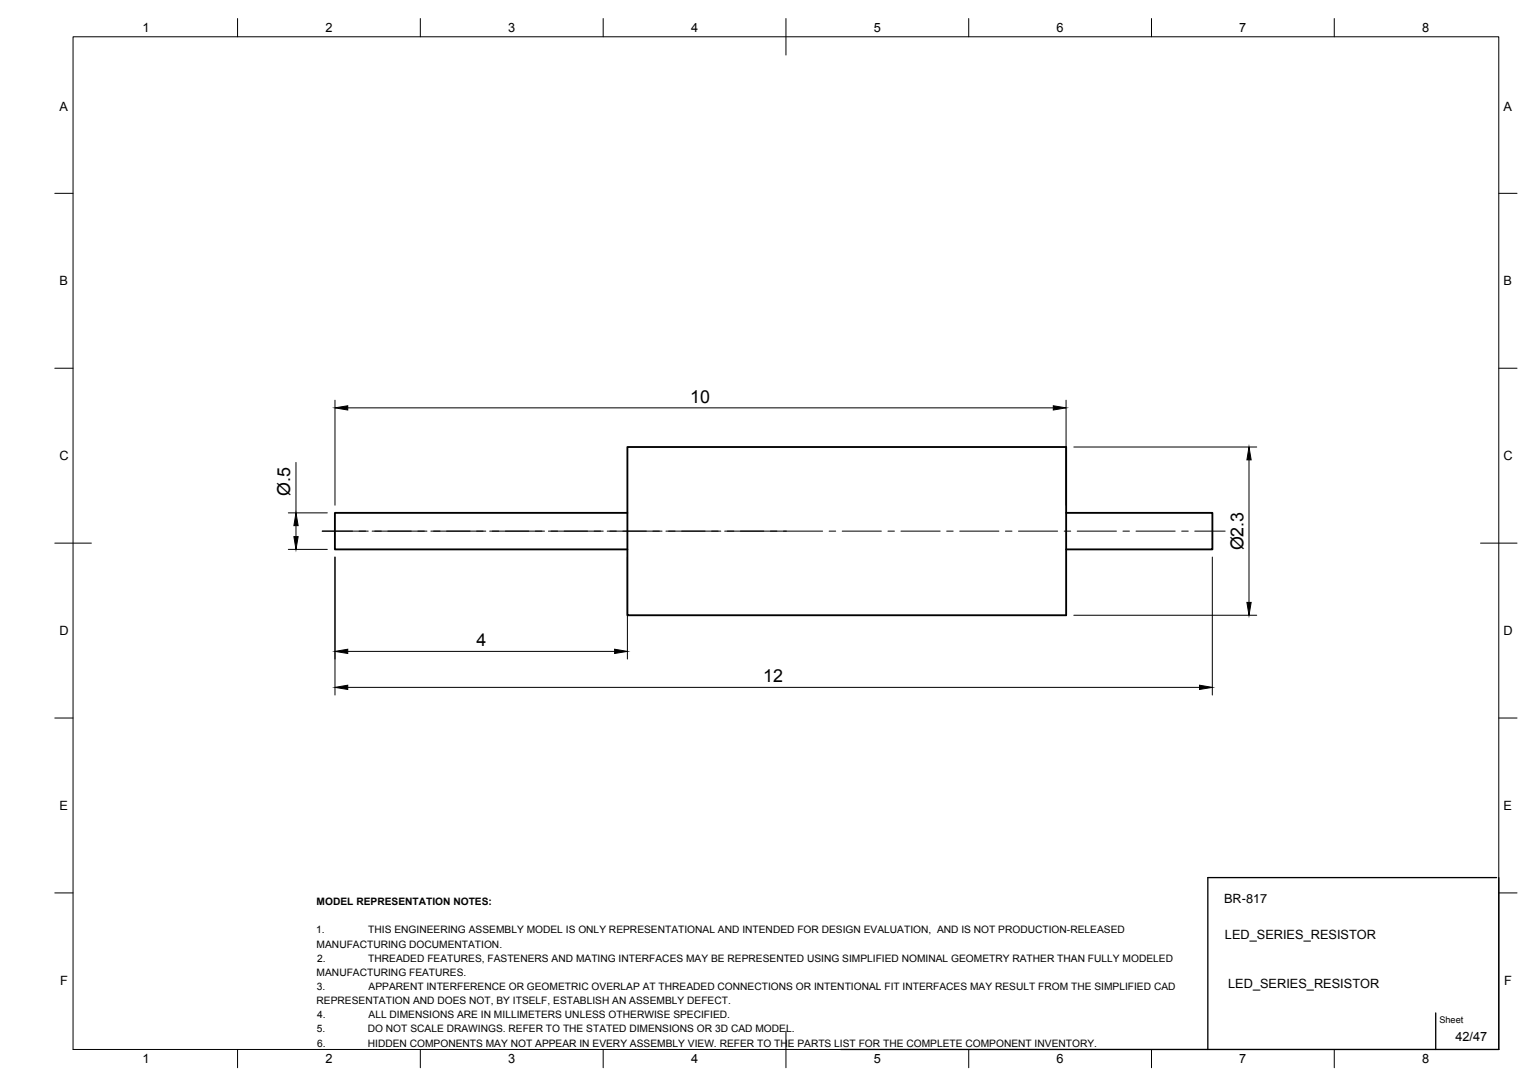
ISO-10303-21;
HEADER;
FILE_DESCRIPTION((''),'2;1');
FILE_NAME('LED_SERIES_RESISTOR.step','2026-10-01T22:07:29-07:00',(''),(''),'','','');
FILE_SCHEMA (('AUTOMOTIVE_DESIGN { 1 0 10303 214 3 1 1 }'));
ENDSEC;
DATA;
#10=MECHANICAL_DESIGN_GEOMETRIC_PRESENTATION_REPRESENTATION('',(#575,#576,#577),#15484);
#502=SHAPE_REPRESENTATION_RELATIONSHIP('SRR','None',#15653,#537) ;
#537=ADVANCED_BREP_SHAPE_REPRESENTATION('',(#616,#617,#618),#15477) ;
#575=STYLED_ITEM('',(#15833),#616) ;
#576=STYLED_ITEM('',(#15842),#617) ;
#577=STYLED_ITEM('',(#15842),#618) ;
#616=MANIFOLD_SOLID_BREP('RESISTOR_BODY',#8286) ;
#617=MANIFOLD_SOLID_BREP('RESISTOR_LEADS',#8287) ;
#618=MANIFOLD_SOLID_BREP('RESISTOR_LEADS',#8288) ;
#798=CYLINDRICAL_SURFACE('',#9829,0.115) ;
#799=CYLINDRICAL_SURFACE('',#9834,0.025) ;
#800=CYLINDRICAL_SURFACE('',#9839,0.025) ;
#1337=CIRCLE('',#9830,0.115) ;
#1338=CIRCLE('',#9831,0.115) ;
#1339=CIRCLE('',#9835,0.025) ;
#1340=CIRCLE('',#9836,0.025) ;
#1341=CIRCLE('',#9840,0.025) ;
#1342=CIRCLE('',#9841,0.025) ;
#1822=FACE_OUTER_BOUND('',#2393,.T.) ;
#1823=FACE_OUTER_BOUND('',#2394,.T.) ;
#1824=FACE_OUTER_BOUND('',#2395,.T.) ;
#1825=FACE_OUTER_BOUND('',#2396,.T.) ;
#1826=FACE_OUTER_BOUND('',#2397,.T.) ;
#1827=FACE_OUTER_BOUND('',#2398,.T.) ;
#1828=FACE_OUTER_BOUND('',#2399,.T.) ;
#1829=FACE_OUTER_BOUND('',#2400,.T.) ;
#1830=FACE_OUTER_BOUND('',#2401,.T.) ;
#2393=EDGE_LOOP('',(#7399,#7400,#7401,#7402)) ;
#2394=EDGE_LOOP('',(#7403)) ;
#2395=EDGE_LOOP('',(#7404)) ;
#2396=EDGE_LOOP('',(#7405,#7406,#7407,#7408)) ;
#2397=EDGE_LOOP('',(#7409)) ;
#2398=EDGE_LOOP('',(#7410)) ;
#2399=EDGE_LOOP('',(#7411,#7412,#7413,#7414)) ;
#2400=EDGE_LOOP('',(#7415)) ;
#2401=EDGE_LOOP('',(#7416)) ;
#2873=LINE('',#15220,#3347) ;
#2874=LINE('',#15228,#3348) ;
#2875=LINE('',#15236,#3349) ;
#3347=VECTOR('',#12656,0.115) ;
#3348=VECTOR('',#12667,0.025) ;
#3349=VECTOR('',#12678,0.025) ;
#4095=VERTEX_POINT('',#15217) ;
#4096=VERTEX_POINT('',#15219) ;
#4097=VERTEX_POINT('',#15225) ;
#4098=VERTEX_POINT('',#15227) ;
#4099=VERTEX_POINT('',#15233) ;
#4100=VERTEX_POINT('',#15235) ;
#5204=EDGE_CURVE('',#4095,#4095,#1337,.T.) ;
#5205=EDGE_CURVE('',#4095,#4096,#2873,.T.) ;
#5206=EDGE_CURVE('',#4096,#4096,#1338,.T.) ;
#5207=EDGE_CURVE('',#4097,#4097,#1339,.T.) ;
#5208=EDGE_CURVE('',#4097,#4098,#2874,.T.) ;
#5209=EDGE_CURVE('',#4098,#4098,#1340,.T.) ;
#5210=EDGE_CURVE('',#4099,#4099,#1341,.T.) ;
#5211=EDGE_CURVE('',#4099,#4100,#2875,.T.) ;
#5212=EDGE_CURVE('',#4100,#4100,#1342,.T.) ;
#7399=ORIENTED_EDGE('',*,*,#5204,.F.) ;
#7400=ORIENTED_EDGE('',*,*,#5205,.T.) ;
#7401=ORIENTED_EDGE('',*,*,#5206,.F.) ;
#7402=ORIENTED_EDGE('',*,*,#5205,.F.) ;
#7403=ORIENTED_EDGE('',*,*,#5206,.T.) ;
#7404=ORIENTED_EDGE('',*,*,#5204,.T.) ;
#7405=ORIENTED_EDGE('',*,*,#5207,.F.) ;
#7406=ORIENTED_EDGE('',*,*,#5208,.T.) ;
#7407=ORIENTED_EDGE('',*,*,#5209,.F.) ;
#7408=ORIENTED_EDGE('',*,*,#5208,.F.) ;
#7409=ORIENTED_EDGE('',*,*,#5209,.T.) ;
#7410=ORIENTED_EDGE('',*,*,#5207,.T.) ;
#7411=ORIENTED_EDGE('',*,*,#5210,.F.) ;
#7412=ORIENTED_EDGE('',*,*,#5211,.T.) ;
#7413=ORIENTED_EDGE('',*,*,#5212,.F.) ;
#7414=ORIENTED_EDGE('',*,*,#5211,.F.) ;
#7415=ORIENTED_EDGE('',*,*,#5212,.T.) ;
#7416=ORIENTED_EDGE('',*,*,#5210,.T.) ;
#7721=PLANE('',#9832) ;
#7722=PLANE('',#9833) ;
#7723=PLANE('',#9837) ;
#7724=PLANE('',#9838) ;
#7725=PLANE('',#9842) ;
#7726=PLANE('',#9843) ;
#8209=ADVANCED_FACE('',(#1822),#798,.T.) ;
#8210=ADVANCED_FACE('',(#1823),#7721,.T.) ;
#8211=ADVANCED_FACE('',(#1824),#7722,.T.) ;
#8212=ADVANCED_FACE('',(#1825),#799,.T.) ;
#8213=ADVANCED_FACE('',(#1826),#7723,.T.) ;
#8214=ADVANCED_FACE('',(#1827),#7724,.T.) ;
#8215=ADVANCED_FACE('',(#1828),#800,.T.) ;
#8216=ADVANCED_FACE('',(#1829),#7725,.T.) ;
#8217=ADVANCED_FACE('',(#1830),#7726,.T.) ;
#8286=CLOSED_SHELL('',(#8209,#8210,#8211)) ;
#8287=CLOSED_SHELL('',(#8212,#8213,#8214)) ;
#8288=CLOSED_SHELL('',(#8215,#8216,#8217)) ;
#9828=AXIS2_PLACEMENT_3D('',#15215,#12650,#12651) ;
#9829=AXIS2_PLACEMENT_3D('',#15216,#12652,#12653) ;
#9830=AXIS2_PLACEMENT_3D('',#15218,#12654,#12655) ;
#9831=AXIS2_PLACEMENT_3D('',#15221,#12657,#12658) ;
#9832=AXIS2_PLACEMENT_3D('',#15222,#12659,#12660) ;
#9833=AXIS2_PLACEMENT_3D('',#15223,#12661,#12662) ;
#9834=AXIS2_PLACEMENT_3D('',#15224,#12663,#12664) ;
#9835=AXIS2_PLACEMENT_3D('',#15226,#12665,#12666) ;
#9836=AXIS2_PLACEMENT_3D('',#15229,#12668,#12669) ;
#9837=AXIS2_PLACEMENT_3D('',#15230,#12670,#12671) ;
#9838=AXIS2_PLACEMENT_3D('',#15231,#12672,#12673) ;
#9839=AXIS2_PLACEMENT_3D('',#15232,#12674,#12675) ;
#9840=AXIS2_PLACEMENT_3D('',#15234,#12676,#12677) ;
#9841=AXIS2_PLACEMENT_3D('',#15237,#12679,#12680) ;
#9842=AXIS2_PLACEMENT_3D('',#15238,#12681,#12682) ;
#9843=AXIS2_PLACEMENT_3D('',#15239,#12683,#12684) ;
#12650=DIRECTION('axis',(0.,0.,1.)) ;
#12651=DIRECTION('refdir',(1.,0.,0.)) ;
#12652=DIRECTION('center_axis',(1.,0.,0.)) ;
#12653=DIRECTION('ref_axis',(0.,0.,-1.)) ;
#12654=DIRECTION('center_axis',(1.,0.,0.)) ;
#12655=DIRECTION('ref_axis',(0.,0.,-1.)) ;
#12656=DIRECTION('',(-1.,0.,0.)) ;
#12657=DIRECTION('center_axis',(-1.,0.,0.)) ;
#12658=DIRECTION('ref_axis',(0.,0.,-1.)) ;
#12659=DIRECTION('center_axis',(-1.,0.,0.)) ;
#12660=DIRECTION('ref_axis',(0.,0.,1.)) ;
#12661=DIRECTION('center_axis',(1.,0.,0.)) ;
#12662=DIRECTION('ref_axis',(0.,0.,-1.)) ;
#12663=DIRECTION('center_axis',(1.,0.,0.)) ;
#12664=DIRECTION('ref_axis',(0.,0.,-1.)) ;
#12665=DIRECTION('center_axis',(1.,0.,0.)) ;
#12666=DIRECTION('ref_axis',(0.,0.,-1.)) ;
#12667=DIRECTION('',(-1.,0.,0.)) ;
#12668=DIRECTION('center_axis',(-1.,0.,0.)) ;
#12669=DIRECTION('ref_axis',(0.,0.,-1.)) ;
#12670=DIRECTION('center_axis',(-1.,0.,0.)) ;
#12671=DIRECTION('ref_axis',(0.,0.,1.)) ;
#12672=DIRECTION('center_axis',(1.,0.,0.)) ;
#12673=DIRECTION('ref_axis',(0.,0.,-1.)) ;
#12674=DIRECTION('center_axis',(1.,0.,0.)) ;
#12675=DIRECTION('ref_axis',(0.,0.,-1.)) ;
#12676=DIRECTION('center_axis',(1.,0.,0.)) ;
#12677=DIRECTION('ref_axis',(0.,0.,-1.)) ;
#12678=DIRECTION('',(-1.,0.,0.)) ;
#12679=DIRECTION('center_axis',(-1.,0.,0.)) ;
#12680=DIRECTION('ref_axis',(0.,0.,-1.)) ;
#12681=DIRECTION('center_axis',(-1.,0.,0.)) ;
#12682=DIRECTION('ref_axis',(0.,0.,1.)) ;
#12683=DIRECTION('center_axis',(1.,0.,0.)) ;
#12684=DIRECTION('ref_axis',(0.,0.,-1.)) ;
#15215=CARTESIAN_POINT('',(0.,0.,0.)) ;
#15216=CARTESIAN_POINT('Origin',(-1.7,-0.6,0.7)) ;
#15217=CARTESIAN_POINT('',(-1.4,-0.6,0.815)) ;
#15218=CARTESIAN_POINT('Origin',(-1.4,-0.6,0.7)) ;
#15219=CARTESIAN_POINT('',(-2.,-0.6,0.815)) ;
#15220=CARTESIAN_POINT('',(-1.7,-0.6,0.815)) ;
#15221=CARTESIAN_POINT('Origin',(-2.,-0.6,0.7)) ;
#15222=CARTESIAN_POINT('Origin',(-2.,-0.6,0.7)) ;
#15223=CARTESIAN_POINT('Origin',(-1.4,-0.6,0.7)) ;
#15224=CARTESIAN_POINT('Origin',(-2.1,-0.6,0.7)) ;
#15225=CARTESIAN_POINT('',(-2.,-0.6,0.725)) ;
#15226=CARTESIAN_POINT('Origin',(-2.,-0.6,0.7)) ;
#15227=CARTESIAN_POINT('',(-2.2,-0.6,0.725)) ;
#15228=CARTESIAN_POINT('',(-2.1,-0.6,0.725)) ;
#15229=CARTESIAN_POINT('Origin',(-2.2,-0.6,0.7)) ;
#15230=CARTESIAN_POINT('Origin',(-2.2,-0.6,0.7)) ;
#15231=CARTESIAN_POINT('Origin',(-2.,-0.6,0.7)) ;
#15232=CARTESIAN_POINT('Origin',(-1.2,-0.6,0.7)) ;
#15233=CARTESIAN_POINT('',(-1.,-0.6,0.725)) ;
#15234=CARTESIAN_POINT('Origin',(-1.,-0.6,0.7)) ;
#15235=CARTESIAN_POINT('',(-1.4,-0.6,0.725)) ;
#15236=CARTESIAN_POINT('',(-1.2,-0.6,0.725)) ;
#15237=CARTESIAN_POINT('Origin',(-1.4,-0.6,0.7)) ;
#15238=CARTESIAN_POINT('Origin',(-1.4,-0.6,0.7)) ;
#15239=CARTESIAN_POINT('Origin',(-1.,-0.6,0.7)) ;
#15434=UNCERTAINTY_MEASURE_WITH_UNIT(LENGTH_MEASURE(0.001),#15485,
'DISTANCE_ACCURACY_VALUE',
'Maximum model space distance between geometric entities at asserted c
onnectivities') ;
#15441=UNCERTAINTY_MEASURE_WITH_UNIT(LENGTH_MEASURE(0.001),#15485,
'DISTANCE_ACCURACY_VALUE',
'Maximum model space distance between geometric entities at asserted c
onnectivities') ;
#15477=(
GEOMETRIC_REPRESENTATION_CONTEXT(3)
GLOBAL_UNCERTAINTY_ASSIGNED_CONTEXT((#15434))
GLOBAL_UNIT_ASSIGNED_CONTEXT((#15485,#15487,#15488))
REPRESENTATION_CONTEXT('','3D')
) ;
#15484=(
GEOMETRIC_REPRESENTATION_CONTEXT(3)
GLOBAL_UNCERTAINTY_ASSIGNED_CONTEXT((#15441))
GLOBAL_UNIT_ASSIGNED_CONTEXT((#15485,#15487,#15488))
REPRESENTATION_CONTEXT('','3D')
) ;
#15485=(
LENGTH_UNIT()
NAMED_UNIT(*)
SI_UNIT(.CENTI.,.METRE.)
) ;
#15487=(
NAMED_UNIT(*)
PLANE_ANGLE_UNIT()
SI_UNIT($,.RADIAN.)
) ;
#15488=(
NAMED_UNIT(*)
SI_UNIT($,.STERADIAN.)
SOLID_ANGLE_UNIT()
) ;
#15524=SHAPE_DEFINITION_REPRESENTATION(#15592,#15653) ;
#15592=PRODUCT_DEFINITION_SHAPE('',$,#15696) ;
#15653=SHAPE_REPRESENTATION('',(#9828),#15477) ;
#15660=PRODUCT_DEFINITION_CONTEXT('part definition',#15788,'design') ;
#15696=PRODUCT_DEFINITION('LED_SERIES_RESISTOR',
'LED_SERIES_RESISTOR',#15738,#15660) ;
#15738=PRODUCT_DEFINITION_FORMATION('',$,#15825) ;
#15788=APPLICATION_CONTEXT(
'Core Data for Automotive Mechanical Design Process') ;
#15789=PRODUCT_CONTEXT('part definition',#15788,'mechanical') ;
#15825=PRODUCT('LED_SERIES_RESISTOR','LED_SERIES_RESISTOR',$,(#15789)) ;
#15833=PRESENTATION_STYLE_ASSIGNMENT((#15845)) ;
#15842=PRESENTATION_STYLE_ASSIGNMENT((#15854)) ;
#15845=SURFACE_STYLE_USAGE(.BOTH.,#15857) ;
#15854=SURFACE_STYLE_USAGE(.BOTH.,#15866) ;
#15857=SURFACE_SIDE_STYLE('',(#15869)) ;
#15866=SURFACE_SIDE_STYLE('',(#15878)) ;
#15869=SURFACE_STYLE_FILL_AREA(#15881) ;
#15878=SURFACE_STYLE_FILL_AREA(#15890) ;
#15881=FILL_AREA_STYLE('Nylon 6-6 (White)',(#15893)) ;
#15890=FILL_AREA_STYLE('Copper - Polished',(#15902)) ;
#15893=FILL_AREA_STYLE_COLOUR('Nylon 6-6 (White)',#15905) ;
#15902=FILL_AREA_STYLE_COLOUR('Copper - Polished',#15914) ;
#15905=COLOUR_RGB('Nylon 6-6 (White)', 0.31764706, 0.68627451, 0.89019608) ;
#15914=COLOUR_RGB('Copper - Polished', 0.66274510, 0.83137255, 0.94901961) ;
ENDSEC;
END-ISO-10303-21;
